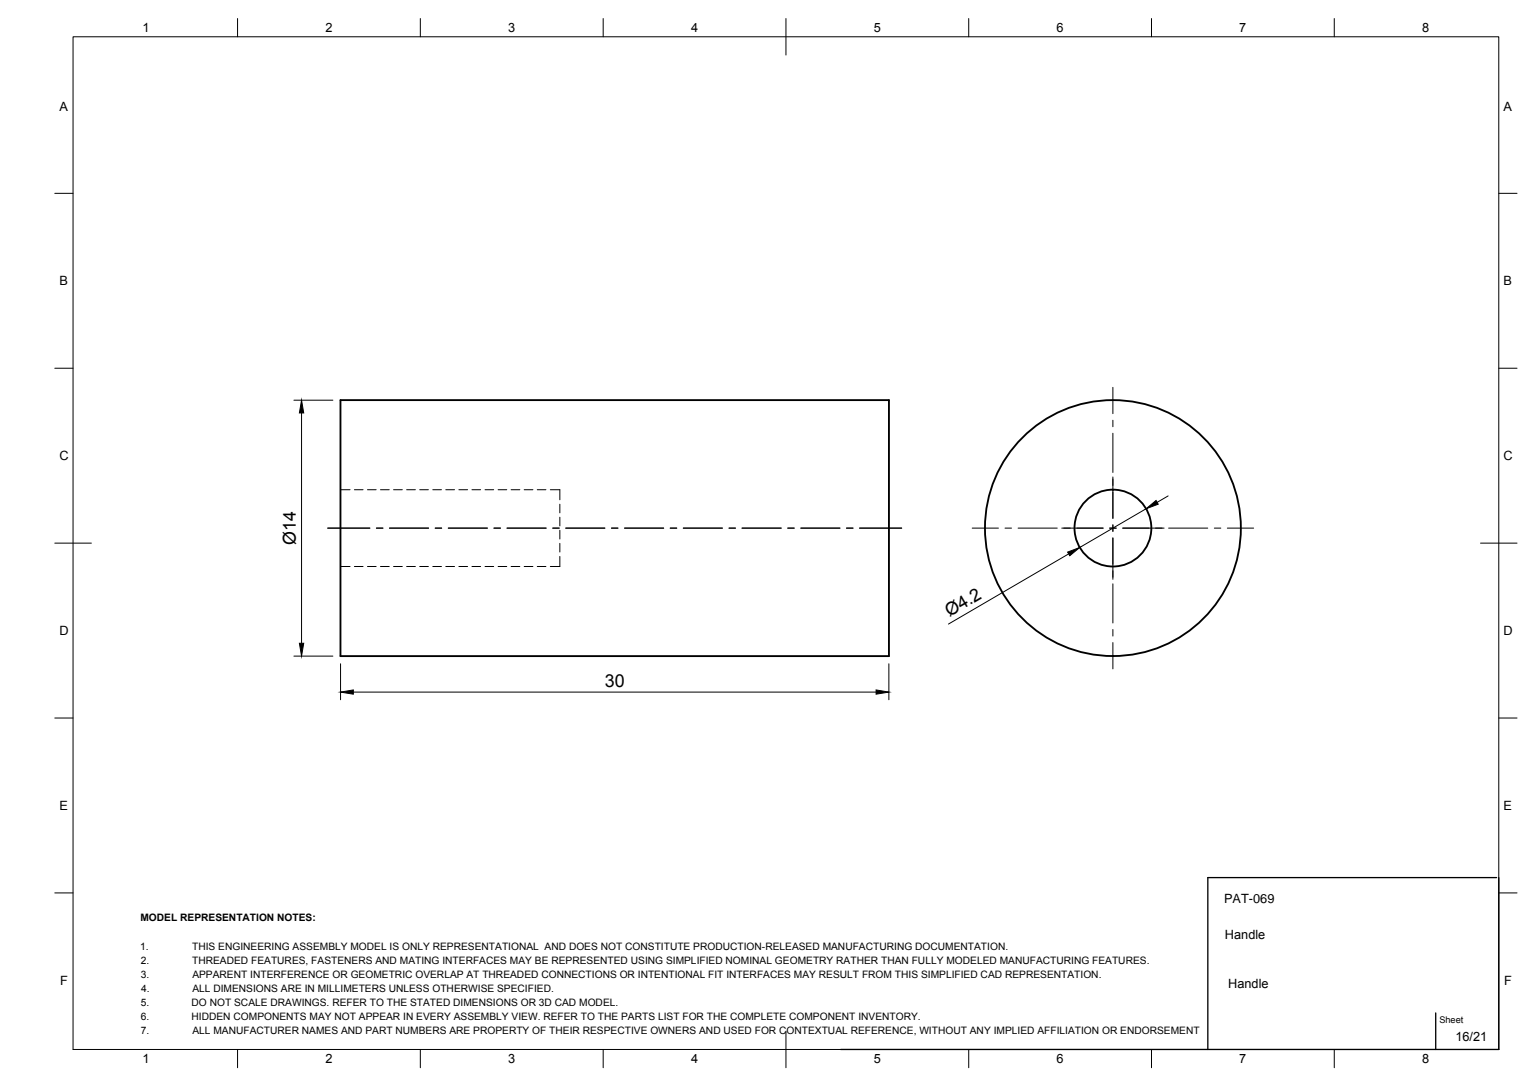
ISO-10303-21;
HEADER;
/* Generated by software containing ST-Developer
 * from STEP Tools, Inc. (www.steptools.com) 
 */

FILE_DESCRIPTION(
/* description */ ('Located fixture plate with toggle clamp'),
/* implementation_level */ '2;1');

FILE_NAME(
/* name */ 'Handle.step',
/* time_stamp */ '2026-10-27T21:36:12-07:00',
/* author */ (''),
/* organization */ (''),
/* preprocessor_version */ 'ST-DEVELOPER v20.2',
/* originating_system */ 'Autodesk Translation Framework v15.17.0.0',
/* authorisation */ '');

FILE_SCHEMA (('AUTOMOTIVE_DESIGN { 1 0 10303 214 3 1 1 }'));
ENDSEC;

DATA;
#10=MECHANICAL_DESIGN_GEOMETRIC_PRESENTATION_REPRESENTATION('',(#334),#9285);
#286=SHAPE_REPRESENTATION_RELATIONSHIP('SRR','None',#9410,#310);
#310=ADVANCED_BREP_SHAPE_REPRESENTATION('',(#356),#9272);
#334=STYLED_ITEM('',(#9605),#356);
#356=MANIFOLD_SOLID_BREP('Body1',#5184);
#464=FACE_BOUND('',#1273,.T.);
#614=PLANE('',#5826);
#615=PLANE('',#5830);
#616=PLANE('',#5831);
#876=FACE_OUTER_BOUND('',#1269,.T.);
#877=FACE_OUTER_BOUND('',#1270,.T.);
#878=FACE_OUTER_BOUND('',#1271,.T.);
#879=FACE_OUTER_BOUND('',#1272,.T.);
#880=FACE_OUTER_BOUND('',#1274,.T.);
#1269=EDGE_LOOP('',(#4426,#4427,#4428,#4429));
#1270=EDGE_LOOP('',(#4430));
#1271=EDGE_LOOP('',(#4431,#4432,#4433,#4434));
#1272=EDGE_LOOP('',(#4435));
#1273=EDGE_LOOP('',(#4436));
#1274=EDGE_LOOP('',(#4437));
#1525=CIRCLE('',#5824,0.21);
#1526=CIRCLE('',#5825,0.21);
#1527=CIRCLE('',#5828,0.7);
#1528=CIRCLE('',#5829,0.7);
#1888=LINE('',#8624,#2298);
#1889=LINE('',#8631,#2299);
#2298=VECTOR('',#7064,0.21);
#2299=VECTOR('',#7073,0.7);
#2711=VERTEX_POINT('',#8621);
#2712=VERTEX_POINT('',#8623);
#2713=VERTEX_POINT('',#8628);
#2714=VERTEX_POINT('',#8630);
#3301=EDGE_CURVE('',#2711,#2711,#1525,.T.);
#3302=EDGE_CURVE('',#2711,#2712,#1888,.T.);
#3303=EDGE_CURVE('',#2712,#2712,#1526,.T.);
#3304=EDGE_CURVE('',#2713,#2713,#1527,.T.);
#3305=EDGE_CURVE('',#2713,#2714,#1889,.T.);
#3306=EDGE_CURVE('',#2714,#2714,#1528,.T.);
#4426=ORIENTED_EDGE('',*,*,#3301,.F.);
#4427=ORIENTED_EDGE('',*,*,#3302,.T.);
#4428=ORIENTED_EDGE('',*,*,#3303,.F.);
#4429=ORIENTED_EDGE('',*,*,#3302,.F.);
#4430=ORIENTED_EDGE('',*,*,#3301,.T.);
#4431=ORIENTED_EDGE('',*,*,#3304,.F.);
#4432=ORIENTED_EDGE('',*,*,#3305,.T.);
#4433=ORIENTED_EDGE('',*,*,#3306,.T.);
#4434=ORIENTED_EDGE('',*,*,#3305,.F.);
#4435=ORIENTED_EDGE('',*,*,#3304,.T.);
#4436=ORIENTED_EDGE('',*,*,#3303,.T.);
#4437=ORIENTED_EDGE('',*,*,#3306,.F.);
#4851=CYLINDRICAL_SURFACE('',#5823,0.21);
#4852=CYLINDRICAL_SURFACE('',#5827,0.7);
#5077=ADVANCED_FACE('',(#876),#4851,.F.);
#5078=ADVANCED_FACE('',(#877),#614,.T.);
#5079=ADVANCED_FACE('',(#878),#4852,.T.);
#5080=ADVANCED_FACE('',(#879,#464),#615,.T.);
#5081=ADVANCED_FACE('',(#880),#616,.F.);
#5184=CLOSED_SHELL('',(#5077,#5078,#5079,#5080,#5081));
#5822=AXIS2_PLACEMENT_3D('',#8619,#7058,#7059);
#5823=AXIS2_PLACEMENT_3D('',#8620,#7060,#7061);
#5824=AXIS2_PLACEMENT_3D('',#8622,#7062,#7063);
#5825=AXIS2_PLACEMENT_3D('',#8625,#7065,#7066);
#5826=AXIS2_PLACEMENT_3D('',#8626,#7067,#7068);
#5827=AXIS2_PLACEMENT_3D('',#8627,#7069,#7070);
#5828=AXIS2_PLACEMENT_3D('',#8629,#7071,#7072);
#5829=AXIS2_PLACEMENT_3D('',#8632,#7074,#7075);
#5830=AXIS2_PLACEMENT_3D('',#8633,#7076,#7077);
#5831=AXIS2_PLACEMENT_3D('',#8634,#7078,#7079);
#7058=DIRECTION('axis',(0.,0.,1.));
#7059=DIRECTION('refdir',(1.,0.,0.));
#7060=DIRECTION('center_axis',(0.,1.,0.));
#7061=DIRECTION('ref_axis',(1.,0.,0.));
#7062=DIRECTION('center_axis',(0.,1.,0.));
#7063=DIRECTION('ref_axis',(1.,0.,0.));
#7064=DIRECTION('',(0.,1.,0.));
#7065=DIRECTION('center_axis',(0.,-1.,0.));
#7066=DIRECTION('ref_axis',(1.,0.,0.));
#7067=DIRECTION('center_axis',(0.,1.,0.));
#7068=DIRECTION('ref_axis',(1.,0.,0.));
#7069=DIRECTION('center_axis',(0.,1.,0.));
#7070=DIRECTION('ref_axis',(1.,0.,0.));
#7071=DIRECTION('center_axis',(0.,1.,0.));
#7072=DIRECTION('ref_axis',(1.,0.,0.));
#7073=DIRECTION('',(0.,-1.,0.));
#7074=DIRECTION('center_axis',(0.,1.,0.));
#7075=DIRECTION('ref_axis',(1.,0.,0.));
#7076=DIRECTION('center_axis',(0.,1.,0.));
#7077=DIRECTION('ref_axis',(1.,0.,0.));
#7078=DIRECTION('center_axis',(0.,1.,0.));
#7079=DIRECTION('ref_axis',(1.,0.,0.));
#8619=CARTESIAN_POINT('',(0.,0.,0.));
#8620=CARTESIAN_POINT('Origin',(0.,-7.7,10.03));
#8621=CARTESIAN_POINT('',(-0.21,-7.7,10.03));
#8622=CARTESIAN_POINT('Origin',(0.,-7.7,10.03));
#8623=CARTESIAN_POINT('',(-0.21,-6.5,10.03));
#8624=CARTESIAN_POINT('',(-0.21,-7.7,10.03));
#8625=CARTESIAN_POINT('Origin',(0.,-6.5,10.03));
#8626=CARTESIAN_POINT('Origin',(0.,-7.7,10.03));
#8627=CARTESIAN_POINT('Origin',(0.,-9.5,10.03));
#8628=CARTESIAN_POINT('',(-0.7,-6.5,10.03));
#8629=CARTESIAN_POINT('Origin',(0.,-6.5,10.03));
#8630=CARTESIAN_POINT('',(-0.7,-9.5,10.03));
#8631=CARTESIAN_POINT('',(-0.7,-9.5,10.03));
#8632=CARTESIAN_POINT('Origin',(0.,-9.5,10.03));
#8633=CARTESIAN_POINT('Origin',(0.,-6.5,10.03));
#8634=CARTESIAN_POINT('Origin',(0.,-9.5,10.03));
#9242=UNCERTAINTY_MEASURE_WITH_UNIT(LENGTH_MEASURE(0.001),#9286,
'DISTANCE_ACCURACY_VALUE',
'Maximum model space distance between geometric entities at asserted c
onnectivities');
#9255=UNCERTAINTY_MEASURE_WITH_UNIT(LENGTH_MEASURE(0.001),#9286,
'DISTANCE_ACCURACY_VALUE',
'Maximum model space distance between geometric entities at asserted c
onnectivities');
#9272=(
GEOMETRIC_REPRESENTATION_CONTEXT(3)
GLOBAL_UNCERTAINTY_ASSIGNED_CONTEXT((#9242))
GLOBAL_UNIT_ASSIGNED_CONTEXT((#9286,#9288,#9289))
REPRESENTATION_CONTEXT('','3D')
);
#9285=(
GEOMETRIC_REPRESENTATION_CONTEXT(3)
GLOBAL_UNCERTAINTY_ASSIGNED_CONTEXT((#9255))
GLOBAL_UNIT_ASSIGNED_CONTEXT((#9286,#9288,#9289))
REPRESENTATION_CONTEXT('','3D')
);
#9286=(
LENGTH_UNIT()
NAMED_UNIT(*)
SI_UNIT(.CENTI.,.METRE.)
);
#9288=(
NAMED_UNIT(*)
PLANE_ANGLE_UNIT()
SI_UNIT($,.RADIAN.)
);
#9289=(
NAMED_UNIT(*)
SI_UNIT($,.STERADIAN.)
SOLID_ANGLE_UNIT()
);
#9306=SHAPE_DEFINITION_REPRESENTATION(#9335,#9410);
#9335=PRODUCT_DEFINITION_SHAPE('',$,#9440);
#9410=SHAPE_REPRESENTATION('',(#5822),#9272);
#9423=PRODUCT_DEFINITION_CONTEXT('part definition',#9512,'design');
#9440=PRODUCT_DEFINITION('Handle','Handle',#9469,#9423);
#9469=PRODUCT_DEFINITION_FORMATION('',$,#9530);
#9512=APPLICATION_CONTEXT(
'Core Data for Automotive Mechanical Design Process');
#9513=PRODUCT_CONTEXT('part definition',#9512,'mechanical');
#9530=PRODUCT('Handle','Handle','Handle',(#9513));
#9599=COLOUR_RGB('Sky Blue',0.24,0.69,0.87);
#9600=FILL_AREA_STYLE_COLOUR('',#9599);
#9601=FILL_AREA_STYLE('',(#9600));
#9602=SURFACE_STYLE_FILL_AREA(#9601);
#9603=SURFACE_SIDE_STYLE('',(#9602));
#9604=SURFACE_STYLE_USAGE(.BOTH.,#9603);
#9605=PRESENTATION_STYLE_ASSIGNMENT((#9604));
ENDSEC;
END-ISO-10303-21;
